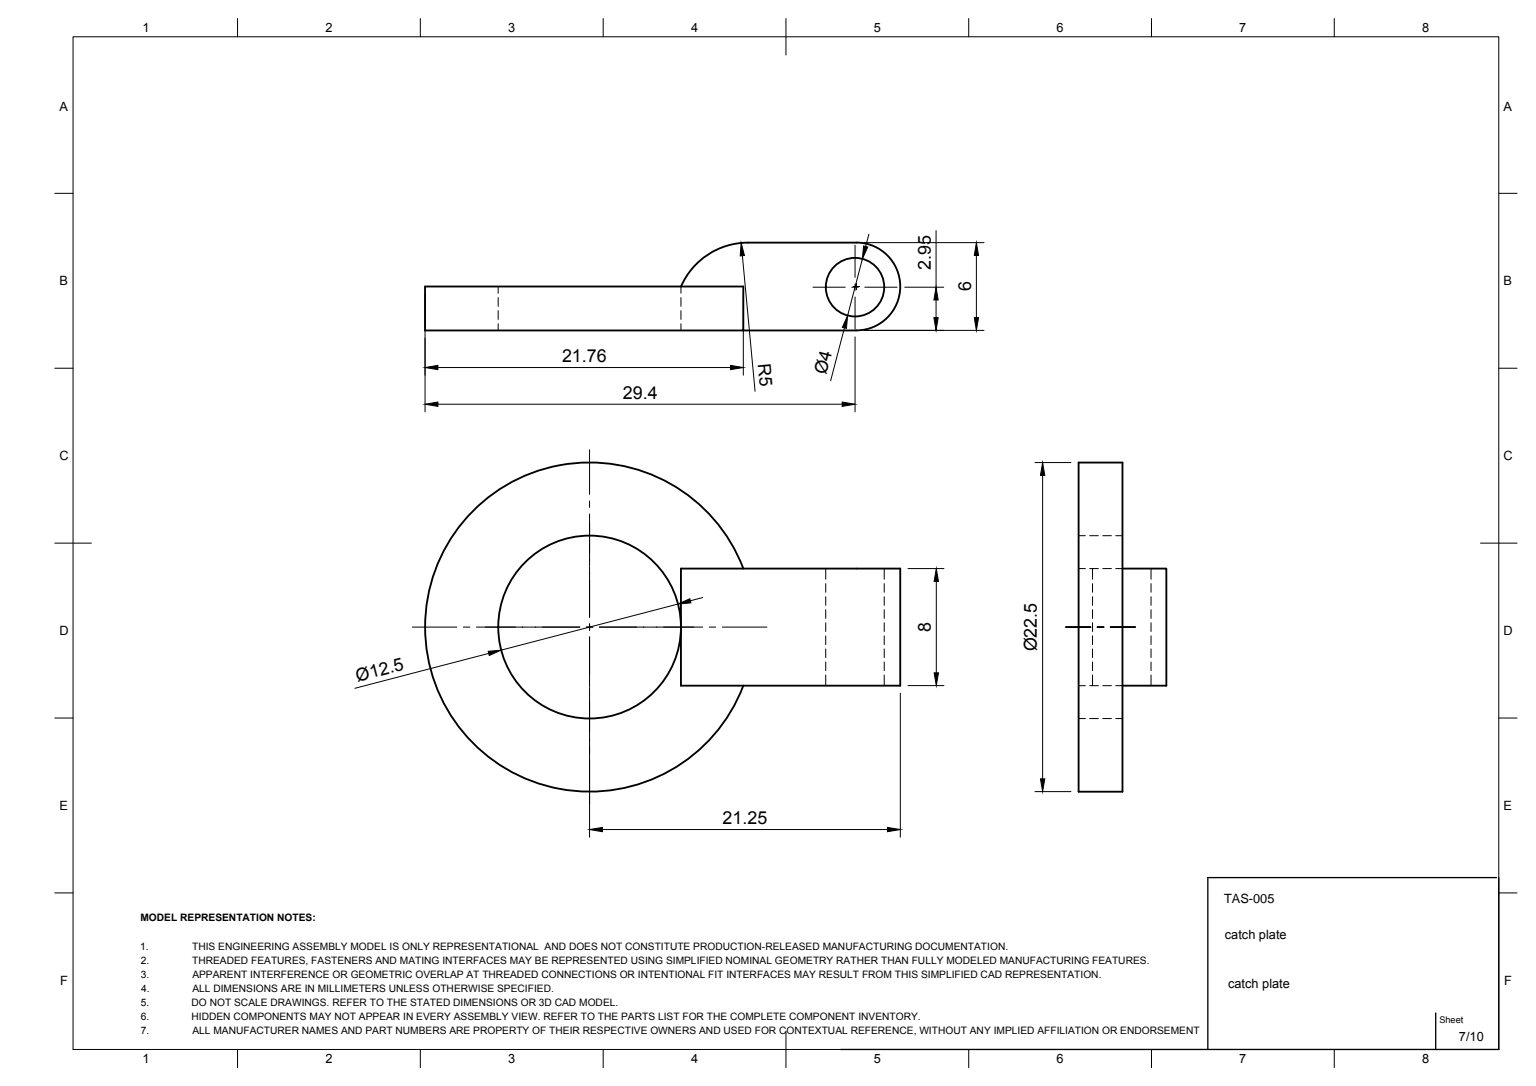
ISO-10303-21;
HEADER;
/* Generated by software containing ST-Developer
 * from STEP Tools, Inc. (www.steptools.com) 
 */

FILE_DESCRIPTION(
/* description */ ('STEP AP214'),
/* implementation_level */ '2;1');

FILE_NAME(
/* name */ 'catch plate.step',
/* time_stamp */ '2026-11-04T19:54:22-08:00',
/* author */ (''),
/* organization */ (''),
/* preprocessor_version */ 'ST-DEVELOPER v20.2',
/* originating_system */ 'Autodesk Translation Framework v15.17.0.0',
/* authorisation */ '');

FILE_SCHEMA (('AUTOMOTIVE_DESIGN { 1 0 10303 214 3 1 1 }'));
ENDSEC;

DATA;
#10=MECHANICAL_DESIGN_GEOMETRIC_PRESENTATION_REPRESENTATION('',(#243),#14084);
#225=SHAPE_REPRESENTATION_RELATIONSHIP('SRR','None',#14124,#234);
#234=ADVANCED_BREP_SHAPE_REPRESENTATION('',(#252),#14079);
#243=STYLED_ITEM('',(#14175),#252);
#252=MANIFOLD_SOLID_BREP('Body1',#3469);
#270=FACE_BOUND('',#697,.T.);
#271=FACE_BOUND('',#699,.T.);
#272=FACE_BOUND('',#701,.T.);
#333=PLANE('',#3752);
#334=PLANE('',#3753);
#335=PLANE('',#3754);
#336=PLANE('',#3757);
#337=PLANE('',#3760);
#489=FACE_OUTER_BOUND('',#692,.T.);
#490=FACE_OUTER_BOUND('',#693,.T.);
#491=FACE_OUTER_BOUND('',#694,.T.);
#492=FACE_OUTER_BOUND('',#695,.T.);
#493=FACE_OUTER_BOUND('',#696,.T.);
#494=FACE_OUTER_BOUND('',#698,.T.);
#495=FACE_OUTER_BOUND('',#700,.T.);
#496=FACE_OUTER_BOUND('',#702,.T.);
#497=FACE_OUTER_BOUND('',#703,.T.);
#498=FACE_OUTER_BOUND('',#704,.T.);
#692=EDGE_LOOP('',(#2883,#2884,#2885,#2886));
#693=EDGE_LOOP('',(#2887,#2888,#2889,#2890,#2891));
#694=EDGE_LOOP('',(#2892,#2893,#2894,#2895));
#695=EDGE_LOOP('',(#2896,#2897,#2898,#2899,#2900,#2901,#2902));
#696=EDGE_LOOP('',(#2903,#2904,#2905,#2906));
#697=EDGE_LOOP('',(#2907));
#698=EDGE_LOOP('',(#2908,#2909,#2910,#2911,#2912,#2913));
#699=EDGE_LOOP('',(#2914));
#700=EDGE_LOOP('',(#2915,#2916,#2917,#2918,#2919,#2920));
#701=EDGE_LOOP('',(#2921));
#702=EDGE_LOOP('',(#2922,#2923,#2924,#2925));
#703=EDGE_LOOP('',(#2926,#2927,#2928,#2929,#2930));
#704=EDGE_LOOP('',(#2931,#2932,#2933,#2934));
#964=LINE('',#9220,#1221);
#965=LINE('',#9227,#1222);
#966=LINE('',#9235,#1223);
#967=LINE('',#9238,#1224);
#968=LINE('',#9241,#1225);
#969=LINE('',#9242,#1226);
#970=LINE('',#9244,#1227);
#971=LINE('',#9245,#1228);
#972=LINE('',#9248,#1229);
#973=LINE('',#9250,#1230);
#974=LINE('',#9251,#1231);
#975=LINE('',#9256,#1232);
#976=LINE('',#9263,#1233);
#977=LINE('',#9265,#1234);
#978=LINE('',#9266,#1235);
#1221=VECTOR('',#4395,2.);
#1222=VECTOR('',#4402,6.25);
#1223=VECTOR('',#4411,1000.);
#1224=VECTOR('',#4414,1000.);
#1225=VECTOR('',#4417,1000.);
#1226=VECTOR('',#4418,1000.);
#1227=VECTOR('',#4419,1000.);
#1228=VECTOR('',#4420,1000.);
#1229=VECTOR('',#4423,1000.);
#1230=VECTOR('',#4424,1000.);
#1231=VECTOR('',#4425,1000.);
#1232=VECTOR('',#4430,1000.);
#1233=VECTOR('',#4439,1000.);
#1234=VECTOR('',#4442,1000.);
#1235=VECTOR('',#4443,1000.);
#1327=CIRCLE('',#3743,2.);
#1328=CIRCLE('',#3744,2.);
#1329=CIRCLE('',#3746,6.25);
#1330=CIRCLE('',#3747,6.25);
#1331=CIRCLE('',#3748,6.25);
#1332=CIRCLE('',#3750,11.25);
#1333=CIRCLE('',#3751,11.25);
#1334=CIRCLE('',#3755,3.);
#1335=CIRCLE('',#3756,5.);
#1336=CIRCLE('',#3758,3.);
#1337=CIRCLE('',#3759,5.);
#1605=VERTEX_POINT('',#9217);
#1606=VERTEX_POINT('',#9219);
#1607=VERTEX_POINT('',#9223);
#1608=VERTEX_POINT('',#9224);
#1609=VERTEX_POINT('',#9226);
#1610=VERTEX_POINT('',#9231);
#1611=VERTEX_POINT('',#9232);
#1612=VERTEX_POINT('',#9234);
#1613=VERTEX_POINT('',#9236);
#1614=VERTEX_POINT('',#9240);
#1615=VERTEX_POINT('',#9243);
#1616=VERTEX_POINT('',#9247);
#1617=VERTEX_POINT('',#9249);
#1618=VERTEX_POINT('',#9253);
#1619=VERTEX_POINT('',#9255);
#1620=VERTEX_POINT('',#9259);
#1621=VERTEX_POINT('',#9261);
#2045=EDGE_CURVE('',#1605,#1605,#1327,.T.);
#2046=EDGE_CURVE('',#1605,#1606,#964,.T.);
#2047=EDGE_CURVE('',#1606,#1606,#1328,.T.);
#2048=EDGE_CURVE('',#1607,#1608,#1329,.T.);
#2049=EDGE_CURVE('',#1608,#1609,#965,.T.);
#2050=EDGE_CURVE('',#1609,#1609,#1330,.T.);
#2051=EDGE_CURVE('',#1608,#1607,#1331,.T.);
#2052=EDGE_CURVE('',#1610,#1611,#1332,.T.);
#2053=EDGE_CURVE('',#1610,#1612,#966,.T.);
#2054=EDGE_CURVE('',#1612,#1613,#1333,.T.);
#2055=EDGE_CURVE('',#1611,#1613,#967,.T.);
#2056=EDGE_CURVE('',#1611,#1614,#968,.T.);
#2057=EDGE_CURVE('',#1607,#1614,#969,.T.);
#2058=EDGE_CURVE('',#1615,#1607,#970,.T.);
#2059=EDGE_CURVE('',#1610,#1615,#971,.T.);
#2060=EDGE_CURVE('',#1612,#1616,#972,.T.);
#2061=EDGE_CURVE('',#1616,#1617,#973,.T.);
#2062=EDGE_CURVE('',#1613,#1617,#974,.T.);
#2063=EDGE_CURVE('',#1617,#1618,#1334,.T.);
#2064=EDGE_CURVE('',#1619,#1618,#975,.T.);
#2065=EDGE_CURVE('',#1619,#1614,#1335,.T.);
#2066=EDGE_CURVE('',#1620,#1616,#1336,.T.);
#2067=EDGE_CURVE('',#1615,#1621,#1337,.T.);
#2068=EDGE_CURVE('',#1621,#1620,#976,.T.);
#2069=EDGE_CURVE('',#1618,#1620,#977,.T.);
#2070=EDGE_CURVE('',#1621,#1619,#978,.T.);
#2883=ORIENTED_EDGE('',*,*,#2045,.T.);
#2884=ORIENTED_EDGE('',*,*,#2046,.T.);
#2885=ORIENTED_EDGE('',*,*,#2047,.F.);
#2886=ORIENTED_EDGE('',*,*,#2046,.F.);
#2887=ORIENTED_EDGE('',*,*,#2048,.T.);
#2888=ORIENTED_EDGE('',*,*,#2049,.T.);
#2889=ORIENTED_EDGE('',*,*,#2050,.F.);
#2890=ORIENTED_EDGE('',*,*,#2049,.F.);
#2891=ORIENTED_EDGE('',*,*,#2051,.T.);
#2892=ORIENTED_EDGE('',*,*,#2052,.F.);
#2893=ORIENTED_EDGE('',*,*,#2053,.T.);
#2894=ORIENTED_EDGE('',*,*,#2054,.T.);
#2895=ORIENTED_EDGE('',*,*,#2055,.F.);
#2896=ORIENTED_EDGE('',*,*,#2052,.T.);
#2897=ORIENTED_EDGE('',*,*,#2056,.T.);
#2898=ORIENTED_EDGE('',*,*,#2057,.F.);
#2899=ORIENTED_EDGE('',*,*,#2051,.F.);
#2900=ORIENTED_EDGE('',*,*,#2048,.F.);
#2901=ORIENTED_EDGE('',*,*,#2058,.F.);
#2902=ORIENTED_EDGE('',*,*,#2059,.F.);
#2903=ORIENTED_EDGE('',*,*,#2060,.T.);
#2904=ORIENTED_EDGE('',*,*,#2061,.T.);
#2905=ORIENTED_EDGE('',*,*,#2062,.F.);
#2906=ORIENTED_EDGE('',*,*,#2054,.F.);
#2907=ORIENTED_EDGE('',*,*,#2050,.T.);
#2908=ORIENTED_EDGE('',*,*,#2062,.T.);
#2909=ORIENTED_EDGE('',*,*,#2063,.T.);
#2910=ORIENTED_EDGE('',*,*,#2064,.F.);
#2911=ORIENTED_EDGE('',*,*,#2065,.T.);
#2912=ORIENTED_EDGE('',*,*,#2056,.F.);
#2913=ORIENTED_EDGE('',*,*,#2055,.T.);
#2914=ORIENTED_EDGE('',*,*,#2047,.T.);
#2915=ORIENTED_EDGE('',*,*,#2066,.T.);
#2916=ORIENTED_EDGE('',*,*,#2060,.F.);
#2917=ORIENTED_EDGE('',*,*,#2053,.F.);
#2918=ORIENTED_EDGE('',*,*,#2059,.T.);
#2919=ORIENTED_EDGE('',*,*,#2067,.T.);
#2920=ORIENTED_EDGE('',*,*,#2068,.T.);
#2921=ORIENTED_EDGE('',*,*,#2045,.F.);
#2922=ORIENTED_EDGE('',*,*,#2064,.T.);
#2923=ORIENTED_EDGE('',*,*,#2069,.T.);
#2924=ORIENTED_EDGE('',*,*,#2068,.F.);
#2925=ORIENTED_EDGE('',*,*,#2070,.T.);
#2926=ORIENTED_EDGE('',*,*,#2065,.F.);
#2927=ORIENTED_EDGE('',*,*,#2070,.F.);
#2928=ORIENTED_EDGE('',*,*,#2067,.F.);
#2929=ORIENTED_EDGE('',*,*,#2058,.T.);
#2930=ORIENTED_EDGE('',*,*,#2057,.T.);
#2931=ORIENTED_EDGE('',*,*,#2066,.F.);
#2932=ORIENTED_EDGE('',*,*,#2069,.F.);
#2933=ORIENTED_EDGE('',*,*,#2063,.F.);
#2934=ORIENTED_EDGE('',*,*,#2061,.F.);
#3259=CYLINDRICAL_SURFACE('',#3742,2.);
#3260=CYLINDRICAL_SURFACE('',#3745,6.25);
#3261=CYLINDRICAL_SURFACE('',#3749,11.25);
#3262=CYLINDRICAL_SURFACE('',#3761,5.);
#3263=CYLINDRICAL_SURFACE('',#3762,3.);
#3399=ADVANCED_FACE('',(#489),#3259,.F.);
#3400=ADVANCED_FACE('',(#490),#3260,.F.);
#3401=ADVANCED_FACE('',(#491),#3261,.T.);
#3402=ADVANCED_FACE('',(#492),#333,.T.);
#3403=ADVANCED_FACE('',(#493,#270),#334,.F.);
#3404=ADVANCED_FACE('',(#494,#271),#335,.F.);
#3405=ADVANCED_FACE('',(#495,#272),#336,.T.);
#3406=ADVANCED_FACE('',(#496),#337,.F.);
#3407=ADVANCED_FACE('',(#497),#3262,.T.);
#3408=ADVANCED_FACE('',(#498),#3263,.T.);
#3469=CLOSED_SHELL('',(#3399,#3400,#3401,#3402,#3403,#3404,#3405,#3406,
#3407,#3408));
#3741=AXIS2_PLACEMENT_3D('',#9215,#4389,#4390);
#3742=AXIS2_PLACEMENT_3D('',#9216,#4391,#4392);
#3743=AXIS2_PLACEMENT_3D('',#9218,#4393,#4394);
#3744=AXIS2_PLACEMENT_3D('',#9221,#4396,#4397);
#3745=AXIS2_PLACEMENT_3D('',#9222,#4398,#4399);
#3746=AXIS2_PLACEMENT_3D('',#9225,#4400,#4401);
#3747=AXIS2_PLACEMENT_3D('',#9228,#4403,#4404);
#3748=AXIS2_PLACEMENT_3D('',#9229,#4405,#4406);
#3749=AXIS2_PLACEMENT_3D('',#9230,#4407,#4408);
#3750=AXIS2_PLACEMENT_3D('',#9233,#4409,#4410);
#3751=AXIS2_PLACEMENT_3D('',#9237,#4412,#4413);
#3752=AXIS2_PLACEMENT_3D('',#9239,#4415,#4416);
#3753=AXIS2_PLACEMENT_3D('',#9246,#4421,#4422);
#3754=AXIS2_PLACEMENT_3D('',#9252,#4426,#4427);
#3755=AXIS2_PLACEMENT_3D('',#9254,#4428,#4429);
#3756=AXIS2_PLACEMENT_3D('',#9257,#4431,#4432);
#3757=AXIS2_PLACEMENT_3D('',#9258,#4433,#4434);
#3758=AXIS2_PLACEMENT_3D('',#9260,#4435,#4436);
#3759=AXIS2_PLACEMENT_3D('',#9262,#4437,#4438);
#3760=AXIS2_PLACEMENT_3D('',#9264,#4440,#4441);
#3761=AXIS2_PLACEMENT_3D('',#9267,#4444,#4445);
#3762=AXIS2_PLACEMENT_3D('',#9268,#4446,#4447);
#4389=DIRECTION('axis',(0.,0.,1.));
#4390=DIRECTION('refdir',(1.,0.,0.));
#4391=DIRECTION('center_axis',(0.,0.,1.));
#4392=DIRECTION('ref_axis',(1.,0.,0.));
#4393=DIRECTION('center_axis',(0.,0.,-1.));
#4394=DIRECTION('ref_axis',(-1.,0.,0.));
#4395=DIRECTION('',(0.,0.,1.));
#4396=DIRECTION('center_axis',(0.,0.,-1.));
#4397=DIRECTION('ref_axis',(-1.,0.,0.));
#4398=DIRECTION('center_axis',(0.,-1.,0.));
#4399=DIRECTION('ref_axis',(0.,0.,-1.));
#4400=DIRECTION('center_axis',(0.,1.,0.));
#4401=DIRECTION('ref_axis',(0.,0.,1.));
#4402=DIRECTION('',(0.,-1.,0.));
#4403=DIRECTION('center_axis',(0.,1.,0.));
#4404=DIRECTION('ref_axis',(0.,0.,1.));
#4405=DIRECTION('center_axis',(0.,1.,0.));
#4406=DIRECTION('ref_axis',(0.,0.,1.));
#4407=DIRECTION('center_axis',(0.,-1.,0.));
#4408=DIRECTION('ref_axis',(-1.,0.,1.83697019872103E-16));
#4409=DIRECTION('center_axis',(0.,1.,0.));
#4410=DIRECTION('ref_axis',(1.,0.,0.));
#4411=DIRECTION('',(0.,-1.,0.));
#4412=DIRECTION('center_axis',(0.,1.,0.));
#4413=DIRECTION('ref_axis',(1.,0.,0.));
#4414=DIRECTION('',(0.,-1.,0.));
#4415=DIRECTION('center_axis',(0.,1.,0.));
#4416=DIRECTION('ref_axis',(0.,0.,1.));
#4417=DIRECTION('',(-1.,0.,0.));
#4418=DIRECTION('',(0.,0.,1.));
#4419=DIRECTION('',(0.,0.,1.));
#4420=DIRECTION('',(-1.,0.,0.));
#4421=DIRECTION('center_axis',(0.,1.,0.));
#4422=DIRECTION('ref_axis',(0.,0.,1.));
#4423=DIRECTION('',(1.,0.,0.));
#4424=DIRECTION('',(0.,0.,1.));
#4425=DIRECTION('',(1.,0.,0.));
#4426=DIRECTION('center_axis',(0.,0.,-1.));
#4427=DIRECTION('ref_axis',(-1.,0.,0.));
#4428=DIRECTION('center_axis',(0.,0.,1.));
#4429=DIRECTION('ref_axis',(-1.,0.,0.));
#4430=DIRECTION('',(1.,0.,0.));
#4431=DIRECTION('center_axis',(0.,0.,1.));
#4432=DIRECTION('ref_axis',(-1.,0.,0.));
#4433=DIRECTION('center_axis',(0.,0.,-1.));
#4434=DIRECTION('ref_axis',(-1.,0.,0.));
#4435=DIRECTION('center_axis',(0.,0.,-1.));
#4436=DIRECTION('ref_axis',(-1.,0.,0.));
#4437=DIRECTION('center_axis',(0.,0.,-1.));
#4438=DIRECTION('ref_axis',(-1.,0.,0.));
#4439=DIRECTION('',(1.,0.,0.));
#4440=DIRECTION('center_axis',(0.,-1.,0.));
#4441=DIRECTION('ref_axis',(-1.,0.,0.));
#4442=DIRECTION('',(0.,0.,-1.));
#4443=DIRECTION('',(0.,0.,1.));
#4444=DIRECTION('center_axis',(0.,0.,-1.));
#4445=DIRECTION('ref_axis',(-1.,0.,0.));
#4446=DIRECTION('center_axis',(0.,0.,-1.));
#4447=DIRECTION('ref_axis',(1.,1.22464679914735E-16,0.));
#9215=CARTESIAN_POINT('',(0.,0.,0.));
#9216=CARTESIAN_POINT('Origin',(18.1535684584702,322.954137916175,6.2));
#9217=CARTESIAN_POINT('',(16.1535684584702,322.954137916175,-4.));
#9218=CARTESIAN_POINT('Origin',(18.1535684584702,322.954137916175,-4.));
#9219=CARTESIAN_POINT('',(16.1535684584702,322.954137916175,4.));
#9220=CARTESIAN_POINT('',(16.1535684584702,322.954137916175,6.2));
#9221=CARTESIAN_POINT('Origin',(18.1535684584702,322.954137916175,4.));
#9222=CARTESIAN_POINT('Origin',(0.,323.,0.));
#9223=CARTESIAN_POINT('',(6.25,323.,0.));
#9224=CARTESIAN_POINT('',(-7.65404249467096E-16,323.,6.25));
#9225=CARTESIAN_POINT('Origin',(0.,323.,0.));
#9226=CARTESIAN_POINT('',(-7.65404249467096E-16,320.,6.25));
#9227=CARTESIAN_POINT('',(-7.65404249467096E-16,323.,6.25));
#9228=CARTESIAN_POINT('Origin',(0.,320.,0.));
#9229=CARTESIAN_POINT('Origin',(0.,323.,0.));
#9230=CARTESIAN_POINT('Origin',(0.,323.,0.));
#9231=CARTESIAN_POINT('',(10.5148704224065,323.,-4.));
#9232=CARTESIAN_POINT('',(10.5148704224065,323.,4.));
#9233=CARTESIAN_POINT('Origin',(0.,323.,0.));
#9234=CARTESIAN_POINT('',(10.5148704224065,320.,-4.));
#9235=CARTESIAN_POINT('',(10.5148704224065,323.,-4.));
#9236=CARTESIAN_POINT('',(10.5148704224065,320.,4.));
#9237=CARTESIAN_POINT('Origin',(0.,320.,0.));
#9238=CARTESIAN_POINT('',(10.5148704224065,323.,4.));
#9239=CARTESIAN_POINT('Origin',(0.,323.,0.));
#9240=CARTESIAN_POINT('',(6.25,323.,4.));
#9241=CARTESIAN_POINT('',(0.,323.,4.));
#9242=CARTESIAN_POINT('',(6.25,323.,0.));
#9243=CARTESIAN_POINT('',(6.25,323.,-4.));
#9244=CARTESIAN_POINT('',(6.25,323.,0.));
#9245=CARTESIAN_POINT('',(0.,323.,-4.));
#9246=CARTESIAN_POINT('Origin',(0.,320.,0.));
#9247=CARTESIAN_POINT('',(18.25,320.,-4.));
#9248=CARTESIAN_POINT('',(6.25,320.,-4.));
#9249=CARTESIAN_POINT('',(18.25,320.,4.));
#9250=CARTESIAN_POINT('',(18.25,320.,4.));
#9251=CARTESIAN_POINT('',(6.25,320.,4.));
#9252=CARTESIAN_POINT('Origin',(6.25,326.,4.));
#9253=CARTESIAN_POINT('',(18.25,326.,4.));
#9254=CARTESIAN_POINT('Origin',(18.25,323.,4.));
#9255=CARTESIAN_POINT('',(10.8325756949558,326.,4.));
#9256=CARTESIAN_POINT('',(6.25,326.,4.));
#9257=CARTESIAN_POINT('Origin',(10.8325756949558,321.,4.));
#9258=CARTESIAN_POINT('Origin',(6.25,326.,-4.));
#9259=CARTESIAN_POINT('',(18.25,326.,-4.));
#9260=CARTESIAN_POINT('Origin',(18.25,323.,-4.));
#9261=CARTESIAN_POINT('',(10.8325756949558,326.,-4.));
#9262=CARTESIAN_POINT('Origin',(10.8325756949558,321.,-4.));
#9263=CARTESIAN_POINT('',(6.25,326.,-4.));
#9264=CARTESIAN_POINT('Origin',(0.,326.,0.));
#9265=CARTESIAN_POINT('',(18.25,326.,-4.));
#9266=CARTESIAN_POINT('',(10.8325756949558,326.,0.));
#9267=CARTESIAN_POINT('Origin',(10.8325756949558,321.,4.));
#9268=CARTESIAN_POINT('Origin',(18.25,323.,-4.));
#14068=UNCERTAINTY_MEASURE_WITH_UNIT(LENGTH_MEASURE(0.01),#14085,
'DISTANCE_ACCURACY_VALUE',
'Maximum model space distance between geometric entities at asserted c
onnectivities');
#14073=UNCERTAINTY_MEASURE_WITH_UNIT(LENGTH_MEASURE(0.01),#14085,
'DISTANCE_ACCURACY_VALUE',
'Maximum model space distance between geometric entities at asserted c
onnectivities');
#14079=(
GEOMETRIC_REPRESENTATION_CONTEXT(3)
GLOBAL_UNCERTAINTY_ASSIGNED_CONTEXT((#14068))
GLOBAL_UNIT_ASSIGNED_CONTEXT((#14085,#14087,#14088))
REPRESENTATION_CONTEXT('','3D')
);
#14084=(
GEOMETRIC_REPRESENTATION_CONTEXT(3)
GLOBAL_UNCERTAINTY_ASSIGNED_CONTEXT((#14073))
GLOBAL_UNIT_ASSIGNED_CONTEXT((#14085,#14087,#14088))
REPRESENTATION_CONTEXT('','3D')
);
#14085=(
LENGTH_UNIT()
NAMED_UNIT(*)
SI_UNIT(.MILLI.,.METRE.)
);
#14087=(
NAMED_UNIT(*)
PLANE_ANGLE_UNIT()
SI_UNIT($,.RADIAN.)
);
#14088=(
NAMED_UNIT(*)
SI_UNIT($,.STERADIAN.)
SOLID_ANGLE_UNIT()
);
#14094=SHAPE_DEFINITION_REPRESENTATION(#14104,#14124);
#14104=PRODUCT_DEFINITION_SHAPE('',$,#14135);
#14124=SHAPE_REPRESENTATION('',(#3741),#14079);
#14129=PRODUCT_DEFINITION_CONTEXT('part definition',#14161,'design');
#14135=PRODUCT_DEFINITION('catch plate','catch plate',#14145,#14129);
#14145=PRODUCT_DEFINITION_FORMATION('',$,#14168);
#14161=APPLICATION_CONTEXT(
'Core Data for Automotive Mechanical Design Process');
#14162=PRODUCT_CONTEXT('part definition',#14161,'mechanical');
#14168=PRODUCT('catch plate','catch plate',$,(#14162));
#14175=PRESENTATION_STYLE_ASSIGNMENT((#14181));
#14181=SURFACE_STYLE_USAGE(.BOTH.,#14187);
#14187=SURFACE_SIDE_STYLE('',(#14193));
#14193=SURFACE_STYLE_FILL_AREA(#14199);
#14199=FILL_AREA_STYLE('Opaque(227,224,212)',(#14205));
#14205=FILL_AREA_STYLE_COLOUR('Opaque(227,224,212)',#14211);
#14211=COLOUR_RGB('Opaque(227,224,212)',0.890196078431372,0.87843137254902,
0.831372549019608);
ENDSEC;
END-ISO-10303-21;
